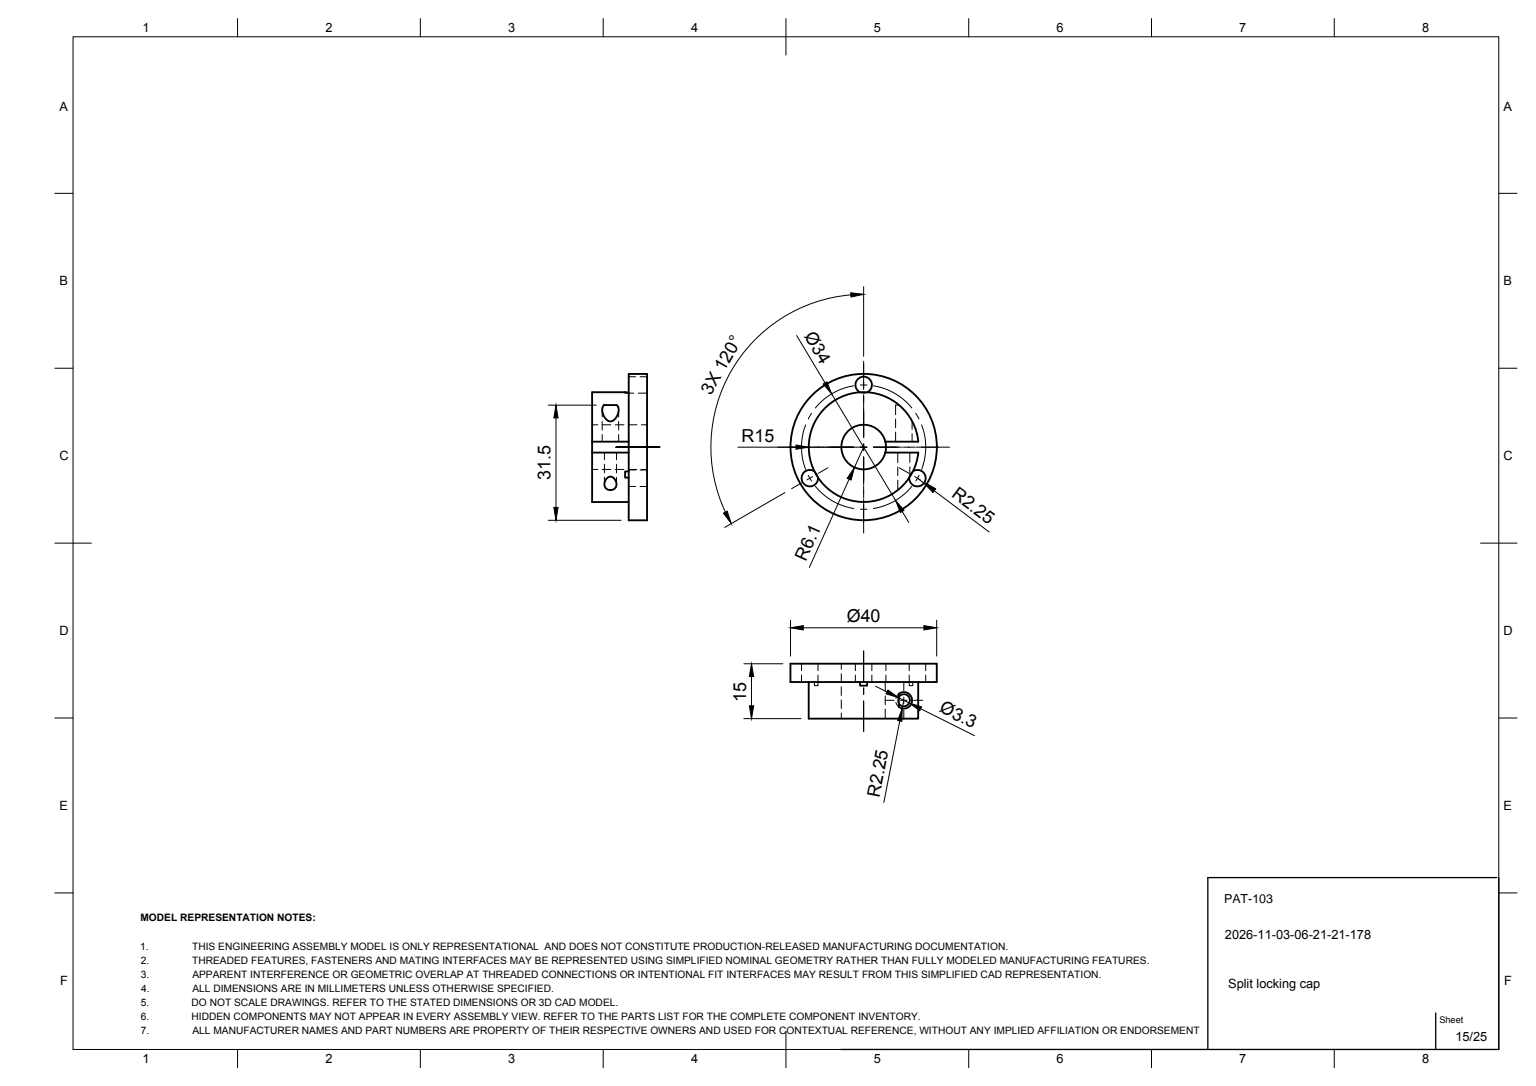
ISO-10303-21;
HEADER;
/* Generated by software containing ST-Developer
 * from STEP Tools, Inc. (www.steptools.com) 
 */

FILE_DESCRIPTION(
/* description */ ('Telescoping shaft support with lock collar'),
/* implementation_level */ '2;1');

FILE_NAME(
/* name */ 'Split locking cap.step',
/* time_stamp */ '2026-10-27T10:48:51-07:00',
/* author */ (''),
/* organization */ (''),
/* preprocessor_version */ 'ST-DEVELOPER v20.2',
/* originating_system */ 'Autodesk Translation Framework v15.17.0.0',
/* authorisation */ '');

FILE_SCHEMA (('AUTOMOTIVE_DESIGN { 1 0 10303 214 3 1 1 }'));
ENDSEC;

DATA;
#10=MECHANICAL_DESIGN_GEOMETRIC_PRESENTATION_REPRESENTATION('',(#251),#7349);
#183=B_SPLINE_CURVE_WITH_KNOTS('',3,(#6551,#6552,#6553,#6554,#6555,#6556,
#6557,#6558),.UNSPECIFIED.,.F.,.F.,(4,2,2,4),(0.211808182408868,0.240806862049815,
0.337801071942656,0.401300756844152),.UNSPECIFIED.);
#184=B_SPLINE_CURVE_WITH_KNOTS('',3,(#6559,#6560,#6561,#6562,#6563,#6564,
#6565,#6566,#6567,#6568,#6569,#6570,#6571,#6572,#6573,#6574,#6575,#6576,
#6577,#6578,#6579,#6580,#6581,#6582,#6583,#6584),.UNSPECIFIED.,.F.,.F.,
(4,2,2,2,2,2,2,2,2,2,2,2,4),(0.401300756844152,0.56115667536452,0.672834477075452,
0.784512278786384,0.830620394066968,0.876728509347553,0.922836624628137,
0.968944739908722,1.08062254161965,1.19230034333059,1.41565594675245,1.51265015664529,
1.54164883628624),.UNSPECIFIED.);
#185=B_SPLINE_CURVE_WITH_KNOTS('',3,(#6588,#6589,#6590,#6591,#6592,#6593,
#6594,#6595,#6596,#6597,#6598,#6599,#6600,#6601,#6602,#6603,#6604,#6605,
#6606,#6607,#6608,#6609,#6610,#6611,#6612,#6613,#6614,#6615,#6616,#6617),
 .UNSPECIFIED.,.F.,.F.,(4,2,2,2,2,2,2,2,2,2,2,2,2,2,4),(0.,0.0607190360347076,
0.121438072069415,0.209441873804407,0.2974456755394,0.399272742727807,0.501099809916215,
0.564787025689956,0.596630633576826,0.628474241463696,0.660317849350566,
0.692161457237437,0.755848673011177,0.857675740199585,0.959502807387993),
 .UNSPECIFIED.);
#186=B_SPLINE_CURVE_WITH_KNOTS('',3,(#6618,#6619,#6620,#6621,#6622,#6623,
#6624,#6625,#6626,#6627),.UNSPECIFIED.,.F.,.F.,(4,2,2,2,4),(0.959502807387993,
1.04750660912298,1.13551041085798,1.19622944689268,1.25694848292739),
 .UNSPECIFIED.);
#211=SHAPE_REPRESENTATION_RELATIONSHIP('SRR','None',#7453,#231);
#231=ADVANCED_BREP_SHAPE_REPRESENTATION('',(#271),#7337);
#251=STYLED_ITEM('',(#7620),#271);
#271=MANIFOLD_SOLID_BREP('Body1',#3974);
#328=FACE_BOUND('',#891,.T.);
#329=FACE_BOUND('',#892,.T.);
#330=FACE_BOUND('',#894,.T.);
#331=FACE_BOUND('',#896,.T.);
#332=FACE_BOUND('',#898,.T.);
#333=FACE_BOUND('',#903,.T.);
#334=FACE_BOUND('',#904,.T.);
#335=FACE_BOUND('',#905,.T.);
#336=FACE_BOUND('',#906,.T.);
#424=PLANE('',#4447);
#425=PLANE('',#4453);
#426=PLANE('',#4460);
#427=PLANE('',#4467);
#428=PLANE('',#4480);
#429=PLANE('',#4481);
#430=PLANE('',#4482);
#431=PLANE('',#4485);
#432=PLANE('',#4492);
#606=FACE_OUTER_BOUND('',#881,.T.);
#607=FACE_OUTER_BOUND('',#882,.T.);
#608=FACE_OUTER_BOUND('',#883,.T.);
#609=FACE_OUTER_BOUND('',#884,.T.);
#610=FACE_OUTER_BOUND('',#885,.T.);
#611=FACE_OUTER_BOUND('',#886,.T.);
#612=FACE_OUTER_BOUND('',#887,.T.);
#613=FACE_OUTER_BOUND('',#888,.T.);
#614=FACE_OUTER_BOUND('',#889,.T.);
#615=FACE_OUTER_BOUND('',#890,.T.);
#616=FACE_OUTER_BOUND('',#893,.T.);
#617=FACE_OUTER_BOUND('',#895,.T.);
#618=FACE_OUTER_BOUND('',#897,.T.);
#619=FACE_OUTER_BOUND('',#899,.T.);
#620=FACE_OUTER_BOUND('',#900,.T.);
#621=FACE_OUTER_BOUND('',#901,.T.);
#622=FACE_OUTER_BOUND('',#902,.T.);
#881=EDGE_LOOP('',(#3158,#3159));
#882=EDGE_LOOP('',(#3160,#3161,#3162,#3163,#3164,#3165));
#883=EDGE_LOOP('',(#3166,#3167,#3168,#3169,#3170));
#884=EDGE_LOOP('',(#3171,#3172));
#885=EDGE_LOOP('',(#3173,#3174,#3175,#3176,#3177,#3178,#3179,#3180));
#886=EDGE_LOOP('',(#3181,#3182));
#887=EDGE_LOOP('',(#3183,#3184,#3185,#3186,#3187,#3188,#3189,#3190));
#888=EDGE_LOOP('',(#3191,#3192));
#889=EDGE_LOOP('',(#3193,#3194,#3195,#3196,#3197,#3198,#3199,#3200));
#890=EDGE_LOOP('',(#3201,#3202,#3203,#3204,#3205,#3206,#3207,#3208,#3209,
#3210,#3211,#3212,#3213,#3214,#3215,#3216));
#891=EDGE_LOOP('',(#3217,#3218,#3219));
#892=EDGE_LOOP('',(#3220,#3221));
#893=EDGE_LOOP('',(#3222,#3223,#3224,#3225));
#894=EDGE_LOOP('',(#3226));
#895=EDGE_LOOP('',(#3227,#3228,#3229,#3230));
#896=EDGE_LOOP('',(#3231));
#897=EDGE_LOOP('',(#3232));
#898=EDGE_LOOP('',(#3233,#3234,#3235,#3236,#3237,#3238,#3239,#3240,#3241,
#3242,#3243,#3244,#3245));
#899=EDGE_LOOP('',(#3246,#3247,#3248,#3249,#3250));
#900=EDGE_LOOP('',(#3251,#3252,#3253,#3254,#3255,#3256,#3257,#3258));
#901=EDGE_LOOP('',(#3259,#3260,#3261,#3262));
#902=EDGE_LOOP('',(#3263));
#903=EDGE_LOOP('',(#3264));
#904=EDGE_LOOP('',(#3265));
#905=EDGE_LOOP('',(#3266));
#906=EDGE_LOOP('',(#3267));
#1169=LINE('',#6544,#1449);
#1170=LINE('',#6550,#1450);
#1171=LINE('',#6629,#1451);
#1172=LINE('',#6640,#1452);
#1173=LINE('',#6643,#1453);
#1174=LINE('',#6645,#1454);
#1175=LINE('',#6656,#1455);
#1176=LINE('',#6659,#1456);
#1177=LINE('',#6661,#1457);
#1178=LINE('',#6672,#1458);
#1179=LINE('',#6675,#1459);
#1180=LINE('',#6677,#1460);
#1181=LINE('',#6685,#1461);
#1182=LINE('',#6689,#1462);
#1183=LINE('',#6694,#1463);
#1184=LINE('',#6695,#1464);
#1185=LINE('',#6696,#1465);
#1186=LINE('',#6700,#1466);
#1187=LINE('',#6701,#1467);
#1188=LINE('',#6702,#1468);
#1189=LINE('',#6713,#1469);
#1190=LINE('',#6717,#1470);
#1449=VECTOR('',#5331,1.);
#1450=VECTOR('',#5338,0.225);
#1451=VECTOR('',#5341,0.164999999999999);
#1452=VECTOR('',#5354,0.225);
#1453=VECTOR('',#5357,1.);
#1454=VECTOR('',#5358,1.);
#1455=VECTOR('',#5371,0.225);
#1456=VECTOR('',#5374,1.);
#1457=VECTOR('',#5375,1.);
#1458=VECTOR('',#5388,0.225);
#1459=VECTOR('',#5391,1.);
#1460=VECTOR('',#5392,1.);
#1461=VECTOR('',#5403,1.);
#1462=VECTOR('',#5406,1.);
#1463=VECTOR('',#5411,1.);
#1464=VECTOR('',#5412,1.);
#1465=VECTOR('',#5413,1.);
#1466=VECTOR('',#5416,1.);
#1467=VECTOR('',#5417,1.);
#1468=VECTOR('',#5418,1.);
#1469=VECTOR('',#5433,0.61);
#1470=VECTOR('',#5438,2.);
#1703=CIRCLE('',#4448,0.225);
#1704=CIRCLE('',#4450,0.225);
#1705=CIRCLE('',#4452,0.164999999999999);
#1706=CIRCLE('',#4454,1.5);
#1707=CIRCLE('',#4455,0.225);
#1708=CIRCLE('',#4457,0.225);
#1709=CIRCLE('',#4458,0.225);
#1710=CIRCLE('',#4459,0.225);
#1711=CIRCLE('',#4461,1.5);
#1712=CIRCLE('',#4462,0.225);
#1713=CIRCLE('',#4464,0.225);
#1714=CIRCLE('',#4465,0.225);
#1715=CIRCLE('',#4466,0.225);
#1716=CIRCLE('',#4468,1.5);
#1717=CIRCLE('',#4469,0.225);
#1718=CIRCLE('',#4471,0.225);
#1719=CIRCLE('',#4472,0.225);
#1720=CIRCLE('',#4473,0.225);
#1721=CIRCLE('',#4475,1.5);
#1722=CIRCLE('',#4476,1.5);
#1723=CIRCLE('',#4477,1.5);
#1724=CIRCLE('',#4478,1.5);
#1725=CIRCLE('',#4479,1.5);
#1726=CIRCLE('',#4483,2.);
#1727=CIRCLE('',#4484,0.61);
#1728=CIRCLE('',#4486,0.61);
#1729=CIRCLE('',#4487,0.61);
#1730=CIRCLE('',#4489,0.61);
#1731=CIRCLE('',#4491,2.);
#1970=VERTEX_POINT('',#6542);
#1971=VERTEX_POINT('',#6543);
#1972=VERTEX_POINT('',#6547);
#1973=VERTEX_POINT('',#6549);
#1974=VERTEX_POINT('',#6586);
#1975=VERTEX_POINT('',#6587);
#1976=VERTEX_POINT('',#6628);
#1977=VERTEX_POINT('',#6632);
#1978=VERTEX_POINT('',#6633);
#1979=VERTEX_POINT('',#6637);
#1980=VERTEX_POINT('',#6639);
#1981=VERTEX_POINT('',#6641);
#1982=VERTEX_POINT('',#6644);
#1983=VERTEX_POINT('',#6648);
#1984=VERTEX_POINT('',#6649);
#1985=VERTEX_POINT('',#6653);
#1986=VERTEX_POINT('',#6655);
#1987=VERTEX_POINT('',#6657);
#1988=VERTEX_POINT('',#6660);
#1989=VERTEX_POINT('',#6664);
#1990=VERTEX_POINT('',#6665);
#1991=VERTEX_POINT('',#6669);
#1992=VERTEX_POINT('',#6671);
#1993=VERTEX_POINT('',#6673);
#1994=VERTEX_POINT('',#6676);
#1995=VERTEX_POINT('',#6682);
#1996=VERTEX_POINT('',#6684);
#1997=VERTEX_POINT('',#6686);
#1998=VERTEX_POINT('',#6688);
#1999=VERTEX_POINT('',#6692);
#2000=VERTEX_POINT('',#6693);
#2001=VERTEX_POINT('',#6698);
#2002=VERTEX_POINT('',#6699);
#2003=VERTEX_POINT('',#6704);
#2004=VERTEX_POINT('',#6708);
#2005=VERTEX_POINT('',#6712);
#2006=VERTEX_POINT('',#6716);
#2391=EDGE_CURVE('',#1970,#1971,#1169,.T.);
#2392=EDGE_CURVE('',#1971,#1970,#1703,.T.);
#2393=EDGE_CURVE('',#1972,#1972,#1704,.T.);
#2394=EDGE_CURVE('',#1972,#1973,#1170,.T.);
#2395=EDGE_CURVE('',#1971,#1973,#183,.T.);
#2396=EDGE_CURVE('',#1973,#1970,#184,.T.);
#2397=EDGE_CURVE('',#1974,#1975,#185,.T.);
#2398=EDGE_CURVE('',#1975,#1974,#186,.T.);
#2399=EDGE_CURVE('',#1975,#1976,#1171,.T.);
#2400=EDGE_CURVE('',#1976,#1976,#1705,.T.);
#2401=EDGE_CURVE('',#1977,#1978,#1706,.T.);
#2402=EDGE_CURVE('',#1978,#1977,#1707,.T.);
#2403=EDGE_CURVE('',#1979,#1979,#1708,.T.);
#2404=EDGE_CURVE('',#1979,#1980,#1172,.T.);
#2405=EDGE_CURVE('',#1981,#1980,#1709,.T.);
#2406=EDGE_CURVE('',#1978,#1981,#1173,.T.);
#2407=EDGE_CURVE('',#1982,#1977,#1174,.T.);
#2408=EDGE_CURVE('',#1980,#1982,#1710,.T.);
#2409=EDGE_CURVE('',#1983,#1984,#1711,.T.);
#2410=EDGE_CURVE('',#1984,#1983,#1712,.T.);
#2411=EDGE_CURVE('',#1985,#1985,#1713,.T.);
#2412=EDGE_CURVE('',#1985,#1986,#1175,.T.);
#2413=EDGE_CURVE('',#1987,#1986,#1714,.T.);
#2414=EDGE_CURVE('',#1984,#1987,#1176,.T.);
#2415=EDGE_CURVE('',#1988,#1983,#1177,.T.);
#2416=EDGE_CURVE('',#1986,#1988,#1715,.T.);
#2417=EDGE_CURVE('',#1989,#1990,#1716,.T.);
#2418=EDGE_CURVE('',#1990,#1989,#1717,.T.);
#2419=EDGE_CURVE('',#1991,#1991,#1718,.T.);
#2420=EDGE_CURVE('',#1991,#1992,#1178,.T.);
#2421=EDGE_CURVE('',#1993,#1992,#1719,.T.);
#2422=EDGE_CURVE('',#1990,#1993,#1179,.T.);
#2423=EDGE_CURVE('',#1994,#1989,#1180,.T.);
#2424=EDGE_CURVE('',#1992,#1994,#1720,.T.);
#2425=EDGE_CURVE('',#1988,#1981,#1721,.T.);
#2426=EDGE_CURVE('',#1994,#1987,#1722,.T.);
#2427=EDGE_CURVE('',#1995,#1993,#1723,.T.);
#2428=EDGE_CURVE('',#1995,#1996,#1181,.T.);
#2429=EDGE_CURVE('',#1997,#1996,#1724,.T.);
#2430=EDGE_CURVE('',#1997,#1998,#1182,.T.);
#2431=EDGE_CURVE('',#1982,#1998,#1725,.T.);
#2432=EDGE_CURVE('',#1999,#2000,#1183,.T.);
#2433=EDGE_CURVE('',#1998,#1999,#1184,.T.);
#2434=EDGE_CURVE('',#2000,#1997,#1185,.T.);
#2435=EDGE_CURVE('',#2001,#2002,#1186,.T.);
#2436=EDGE_CURVE('',#1996,#2001,#1187,.T.);
#2437=EDGE_CURVE('',#2002,#1995,#1188,.T.);
#2438=EDGE_CURVE('',#2003,#2003,#1726,.T.);
#2439=EDGE_CURVE('',#2002,#1999,#1727,.T.);
#2440=EDGE_CURVE('',#2001,#2004,#1728,.T.);
#2441=EDGE_CURVE('',#2004,#2000,#1729,.T.);
#2442=EDGE_CURVE('',#2004,#2005,#1189,.T.);
#2443=EDGE_CURVE('',#2005,#2005,#1730,.T.);
#2444=EDGE_CURVE('',#2003,#2006,#1190,.T.);
#2445=EDGE_CURVE('',#2006,#2006,#1731,.T.);
#3158=ORIENTED_EDGE('',*,*,#2391,.F.);
#3159=ORIENTED_EDGE('',*,*,#2392,.F.);
#3160=ORIENTED_EDGE('',*,*,#2393,.F.);
#3161=ORIENTED_EDGE('',*,*,#2394,.T.);
#3162=ORIENTED_EDGE('',*,*,#2395,.F.);
#3163=ORIENTED_EDGE('',*,*,#2392,.T.);
#3164=ORIENTED_EDGE('',*,*,#2396,.F.);
#3165=ORIENTED_EDGE('',*,*,#2394,.F.);
#3166=ORIENTED_EDGE('',*,*,#2397,.F.);
#3167=ORIENTED_EDGE('',*,*,#2398,.F.);
#3168=ORIENTED_EDGE('',*,*,#2399,.T.);
#3169=ORIENTED_EDGE('',*,*,#2400,.F.);
#3170=ORIENTED_EDGE('',*,*,#2399,.F.);
#3171=ORIENTED_EDGE('',*,*,#2401,.F.);
#3172=ORIENTED_EDGE('',*,*,#2402,.F.);
#3173=ORIENTED_EDGE('',*,*,#2403,.F.);
#3174=ORIENTED_EDGE('',*,*,#2404,.T.);
#3175=ORIENTED_EDGE('',*,*,#2405,.F.);
#3176=ORIENTED_EDGE('',*,*,#2406,.F.);
#3177=ORIENTED_EDGE('',*,*,#2402,.T.);
#3178=ORIENTED_EDGE('',*,*,#2407,.F.);
#3179=ORIENTED_EDGE('',*,*,#2408,.F.);
#3180=ORIENTED_EDGE('',*,*,#2404,.F.);
#3181=ORIENTED_EDGE('',*,*,#2409,.F.);
#3182=ORIENTED_EDGE('',*,*,#2410,.F.);
#3183=ORIENTED_EDGE('',*,*,#2411,.F.);
#3184=ORIENTED_EDGE('',*,*,#2412,.T.);
#3185=ORIENTED_EDGE('',*,*,#2413,.F.);
#3186=ORIENTED_EDGE('',*,*,#2414,.F.);
#3187=ORIENTED_EDGE('',*,*,#2410,.T.);
#3188=ORIENTED_EDGE('',*,*,#2415,.F.);
#3189=ORIENTED_EDGE('',*,*,#2416,.F.);
#3190=ORIENTED_EDGE('',*,*,#2412,.F.);
#3191=ORIENTED_EDGE('',*,*,#2417,.F.);
#3192=ORIENTED_EDGE('',*,*,#2418,.F.);
#3193=ORIENTED_EDGE('',*,*,#2419,.F.);
#3194=ORIENTED_EDGE('',*,*,#2420,.T.);
#3195=ORIENTED_EDGE('',*,*,#2421,.F.);
#3196=ORIENTED_EDGE('',*,*,#2422,.F.);
#3197=ORIENTED_EDGE('',*,*,#2418,.T.);
#3198=ORIENTED_EDGE('',*,*,#2423,.F.);
#3199=ORIENTED_EDGE('',*,*,#2424,.F.);
#3200=ORIENTED_EDGE('',*,*,#2420,.F.);
#3201=ORIENTED_EDGE('',*,*,#2407,.T.);
#3202=ORIENTED_EDGE('',*,*,#2401,.T.);
#3203=ORIENTED_EDGE('',*,*,#2406,.T.);
#3204=ORIENTED_EDGE('',*,*,#2425,.F.);
#3205=ORIENTED_EDGE('',*,*,#2415,.T.);
#3206=ORIENTED_EDGE('',*,*,#2409,.T.);
#3207=ORIENTED_EDGE('',*,*,#2414,.T.);
#3208=ORIENTED_EDGE('',*,*,#2426,.F.);
#3209=ORIENTED_EDGE('',*,*,#2423,.T.);
#3210=ORIENTED_EDGE('',*,*,#2417,.T.);
#3211=ORIENTED_EDGE('',*,*,#2422,.T.);
#3212=ORIENTED_EDGE('',*,*,#2427,.F.);
#3213=ORIENTED_EDGE('',*,*,#2428,.T.);
#3214=ORIENTED_EDGE('',*,*,#2429,.F.);
#3215=ORIENTED_EDGE('',*,*,#2430,.T.);
#3216=ORIENTED_EDGE('',*,*,#2431,.F.);
#3217=ORIENTED_EDGE('',*,*,#2395,.T.);
#3218=ORIENTED_EDGE('',*,*,#2396,.T.);
#3219=ORIENTED_EDGE('',*,*,#2391,.T.);
#3220=ORIENTED_EDGE('',*,*,#2397,.T.);
#3221=ORIENTED_EDGE('',*,*,#2398,.T.);
#3222=ORIENTED_EDGE('',*,*,#2432,.F.);
#3223=ORIENTED_EDGE('',*,*,#2433,.F.);
#3224=ORIENTED_EDGE('',*,*,#2430,.F.);
#3225=ORIENTED_EDGE('',*,*,#2434,.F.);
#3226=ORIENTED_EDGE('',*,*,#2393,.T.);
#3227=ORIENTED_EDGE('',*,*,#2435,.F.);
#3228=ORIENTED_EDGE('',*,*,#2436,.F.);
#3229=ORIENTED_EDGE('',*,*,#2428,.F.);
#3230=ORIENTED_EDGE('',*,*,#2437,.F.);
#3231=ORIENTED_EDGE('',*,*,#2400,.T.);
#3232=ORIENTED_EDGE('',*,*,#2438,.T.);
#3233=ORIENTED_EDGE('',*,*,#2405,.T.);
#3234=ORIENTED_EDGE('',*,*,#2408,.T.);
#3235=ORIENTED_EDGE('',*,*,#2431,.T.);
#3236=ORIENTED_EDGE('',*,*,#2433,.T.);
#3237=ORIENTED_EDGE('',*,*,#2439,.F.);
#3238=ORIENTED_EDGE('',*,*,#2437,.T.);
#3239=ORIENTED_EDGE('',*,*,#2427,.T.);
#3240=ORIENTED_EDGE('',*,*,#2421,.T.);
#3241=ORIENTED_EDGE('',*,*,#2424,.T.);
#3242=ORIENTED_EDGE('',*,*,#2426,.T.);
#3243=ORIENTED_EDGE('',*,*,#2413,.T.);
#3244=ORIENTED_EDGE('',*,*,#2416,.T.);
#3245=ORIENTED_EDGE('',*,*,#2425,.T.);
#3246=ORIENTED_EDGE('',*,*,#2434,.T.);
#3247=ORIENTED_EDGE('',*,*,#2429,.T.);
#3248=ORIENTED_EDGE('',*,*,#2436,.T.);
#3249=ORIENTED_EDGE('',*,*,#2440,.T.);
#3250=ORIENTED_EDGE('',*,*,#2441,.T.);
#3251=ORIENTED_EDGE('',*,*,#2432,.T.);
#3252=ORIENTED_EDGE('',*,*,#2441,.F.);
#3253=ORIENTED_EDGE('',*,*,#2442,.T.);
#3254=ORIENTED_EDGE('',*,*,#2443,.T.);
#3255=ORIENTED_EDGE('',*,*,#2442,.F.);
#3256=ORIENTED_EDGE('',*,*,#2440,.F.);
#3257=ORIENTED_EDGE('',*,*,#2435,.T.);
#3258=ORIENTED_EDGE('',*,*,#2439,.T.);
#3259=ORIENTED_EDGE('',*,*,#2438,.F.);
#3260=ORIENTED_EDGE('',*,*,#2444,.T.);
#3261=ORIENTED_EDGE('',*,*,#2445,.T.);
#3262=ORIENTED_EDGE('',*,*,#2444,.F.);
#3263=ORIENTED_EDGE('',*,*,#2445,.F.);
#3264=ORIENTED_EDGE('',*,*,#2403,.T.);
#3265=ORIENTED_EDGE('',*,*,#2411,.T.);
#3266=ORIENTED_EDGE('',*,*,#2419,.T.);
#3267=ORIENTED_EDGE('',*,*,#2443,.F.);
#3706=CYLINDRICAL_SURFACE('',#4449,0.225);
#3707=CYLINDRICAL_SURFACE('',#4451,0.164999999999999);
#3708=CYLINDRICAL_SURFACE('',#4456,0.225);
#3709=CYLINDRICAL_SURFACE('',#4463,0.225);
#3710=CYLINDRICAL_SURFACE('',#4470,0.225);
#3711=CYLINDRICAL_SURFACE('',#4474,1.5);
#3712=CYLINDRICAL_SURFACE('',#4488,0.61);
#3713=CYLINDRICAL_SURFACE('',#4490,2.);
#3849=ADVANCED_FACE('',(#606),#424,.F.);
#3850=ADVANCED_FACE('',(#607),#3706,.F.);
#3851=ADVANCED_FACE('',(#608),#3707,.F.);
#3852=ADVANCED_FACE('',(#609),#425,.F.);
#3853=ADVANCED_FACE('',(#610),#3708,.F.);
#3854=ADVANCED_FACE('',(#611),#426,.F.);
#3855=ADVANCED_FACE('',(#612),#3709,.F.);
#3856=ADVANCED_FACE('',(#613),#427,.F.);
#3857=ADVANCED_FACE('',(#614),#3710,.F.);
#3858=ADVANCED_FACE('',(#615,#328,#329),#3711,.T.);
#3859=ADVANCED_FACE('',(#616,#330),#428,.F.);
#3860=ADVANCED_FACE('',(#617,#331),#429,.F.);
#3861=ADVANCED_FACE('',(#618,#332),#430,.T.);
#3862=ADVANCED_FACE('',(#619),#431,.T.);
#3863=ADVANCED_FACE('',(#620),#3712,.F.);
#3864=ADVANCED_FACE('',(#621),#3713,.T.);
#3865=ADVANCED_FACE('',(#622,#333,#334,#335,#336),#432,.F.);
#3974=CLOSED_SHELL('',(#3849,#3850,#3851,#3852,#3853,#3854,#3855,#3856,
#3857,#3858,#3859,#3860,#3861,#3862,#3863,#3864,#3865));
#4446=AXIS2_PLACEMENT_3D('',#6540,#5327,#5328);
#4447=AXIS2_PLACEMENT_3D('',#6541,#5329,#5330);
#4448=AXIS2_PLACEMENT_3D('',#6545,#5332,#5333);
#4449=AXIS2_PLACEMENT_3D('',#6546,#5334,#5335);
#4450=AXIS2_PLACEMENT_3D('',#6548,#5336,#5337);
#4451=AXIS2_PLACEMENT_3D('',#6585,#5339,#5340);
#4452=AXIS2_PLACEMENT_3D('',#6630,#5342,#5343);
#4453=AXIS2_PLACEMENT_3D('',#6631,#5344,#5345);
#4454=AXIS2_PLACEMENT_3D('',#6634,#5346,#5347);
#4455=AXIS2_PLACEMENT_3D('',#6635,#5348,#5349);
#4456=AXIS2_PLACEMENT_3D('',#6636,#5350,#5351);
#4457=AXIS2_PLACEMENT_3D('',#6638,#5352,#5353);
#4458=AXIS2_PLACEMENT_3D('',#6642,#5355,#5356);
#4459=AXIS2_PLACEMENT_3D('',#6646,#5359,#5360);
#4460=AXIS2_PLACEMENT_3D('',#6647,#5361,#5362);
#4461=AXIS2_PLACEMENT_3D('',#6650,#5363,#5364);
#4462=AXIS2_PLACEMENT_3D('',#6651,#5365,#5366);
#4463=AXIS2_PLACEMENT_3D('',#6652,#5367,#5368);
#4464=AXIS2_PLACEMENT_3D('',#6654,#5369,#5370);
#4465=AXIS2_PLACEMENT_3D('',#6658,#5372,#5373);
#4466=AXIS2_PLACEMENT_3D('',#6662,#5376,#5377);
#4467=AXIS2_PLACEMENT_3D('',#6663,#5378,#5379);
#4468=AXIS2_PLACEMENT_3D('',#6666,#5380,#5381);
#4469=AXIS2_PLACEMENT_3D('',#6667,#5382,#5383);
#4470=AXIS2_PLACEMENT_3D('',#6668,#5384,#5385);
#4471=AXIS2_PLACEMENT_3D('',#6670,#5386,#5387);
#4472=AXIS2_PLACEMENT_3D('',#6674,#5389,#5390);
#4473=AXIS2_PLACEMENT_3D('',#6678,#5393,#5394);
#4474=AXIS2_PLACEMENT_3D('',#6679,#5395,#5396);
#4475=AXIS2_PLACEMENT_3D('',#6680,#5397,#5398);
#4476=AXIS2_PLACEMENT_3D('',#6681,#5399,#5400);
#4477=AXIS2_PLACEMENT_3D('',#6683,#5401,#5402);
#4478=AXIS2_PLACEMENT_3D('',#6687,#5404,#5405);
#4479=AXIS2_PLACEMENT_3D('',#6690,#5407,#5408);
#4480=AXIS2_PLACEMENT_3D('',#6691,#5409,#5410);
#4481=AXIS2_PLACEMENT_3D('',#6697,#5414,#5415);
#4482=AXIS2_PLACEMENT_3D('',#6703,#5419,#5420);
#4483=AXIS2_PLACEMENT_3D('',#6705,#5421,#5422);
#4484=AXIS2_PLACEMENT_3D('',#6706,#5423,#5424);
#4485=AXIS2_PLACEMENT_3D('',#6707,#5425,#5426);
#4486=AXIS2_PLACEMENT_3D('',#6709,#5427,#5428);
#4487=AXIS2_PLACEMENT_3D('',#6710,#5429,#5430);
#4488=AXIS2_PLACEMENT_3D('',#6711,#5431,#5432);
#4489=AXIS2_PLACEMENT_3D('',#6714,#5434,#5435);
#4490=AXIS2_PLACEMENT_3D('',#6715,#5436,#5437);
#4491=AXIS2_PLACEMENT_3D('',#6718,#5439,#5440);
#4492=AXIS2_PLACEMENT_3D('',#6719,#5441,#5442);
#5327=DIRECTION('axis',(0.,0.,1.));
#5328=DIRECTION('refdir',(1.,0.,0.));
#5329=DIRECTION('center_axis',(0.,0.,1.));
#5330=DIRECTION('ref_axis',(1.,0.,0.));
#5331=DIRECTION('',(-1.,0.,0.));
#5332=DIRECTION('center_axis',(0.,0.,1.));
#5333=DIRECTION('ref_axis',(1.,0.,0.));
#5334=DIRECTION('center_axis',(0.,0.,1.));
#5335=DIRECTION('ref_axis',(1.,0.,0.));
#5336=DIRECTION('center_axis',(0.,0.,1.));
#5337=DIRECTION('ref_axis',(1.,0.,0.));
#5338=DIRECTION('',(0.,0.,1.));
#5339=DIRECTION('center_axis',(0.,0.,1.));
#5340=DIRECTION('ref_axis',(1.,0.,0.));
#5341=DIRECTION('',(0.,0.,1.));
#5342=DIRECTION('center_axis',(0.,0.,-1.));
#5343=DIRECTION('ref_axis',(1.,0.,0.));
#5344=DIRECTION('center_axis',(1.,0.,0.));
#5345=DIRECTION('ref_axis',(0.,0.,-1.));
#5346=DIRECTION('center_axis',(1.,0.,0.));
#5347=DIRECTION('ref_axis',(0.,0.,-1.));
#5348=DIRECTION('center_axis',(1.,0.,0.));
#5349=DIRECTION('ref_axis',(0.,0.,-1.));
#5350=DIRECTION('center_axis',(1.,0.,0.));
#5351=DIRECTION('ref_axis',(0.,0.,-1.));
#5352=DIRECTION('center_axis',(1.,0.,0.));
#5353=DIRECTION('ref_axis',(0.,0.,-1.));
#5354=DIRECTION('',(1.,0.,0.));
#5355=DIRECTION('center_axis',(-1.,0.,0.));
#5356=DIRECTION('ref_axis',(0.,0.,-1.));
#5357=DIRECTION('',(-1.,0.,0.));
#5358=DIRECTION('',(1.,0.,0.));
#5359=DIRECTION('center_axis',(-1.,0.,0.));
#5360=DIRECTION('ref_axis',(0.,0.,-1.));
#5361=DIRECTION('center_axis',(1.,0.,0.));
#5362=DIRECTION('ref_axis',(0.,0.,-1.));
#5363=DIRECTION('center_axis',(1.,0.,0.));
#5364=DIRECTION('ref_axis',(0.,0.,-1.));
#5365=DIRECTION('center_axis',(1.,0.,0.));
#5366=DIRECTION('ref_axis',(0.,0.,-1.));
#5367=DIRECTION('center_axis',(1.,0.,0.));
#5368=DIRECTION('ref_axis',(0.,0.,-1.));
#5369=DIRECTION('center_axis',(1.,0.,0.));
#5370=DIRECTION('ref_axis',(0.,0.,-1.));
#5371=DIRECTION('',(1.,0.,0.));
#5372=DIRECTION('center_axis',(-1.,0.,0.));
#5373=DIRECTION('ref_axis',(0.,0.,-1.));
#5374=DIRECTION('',(-1.,0.,0.));
#5375=DIRECTION('',(1.,0.,0.));
#5376=DIRECTION('center_axis',(-1.,0.,0.));
#5377=DIRECTION('ref_axis',(0.,0.,-1.));
#5378=DIRECTION('center_axis',(1.,0.,0.));
#5379=DIRECTION('ref_axis',(0.,0.,-1.));
#5380=DIRECTION('center_axis',(1.,0.,0.));
#5381=DIRECTION('ref_axis',(0.,0.,-1.));
#5382=DIRECTION('center_axis',(1.,0.,0.));
#5383=DIRECTION('ref_axis',(0.,0.,-1.));
#5384=DIRECTION('center_axis',(1.,0.,0.));
#5385=DIRECTION('ref_axis',(0.,0.,-1.));
#5386=DIRECTION('center_axis',(1.,0.,0.));
#5387=DIRECTION('ref_axis',(0.,0.,-1.));
#5388=DIRECTION('',(1.,0.,0.));
#5389=DIRECTION('center_axis',(-1.,0.,0.));
#5390=DIRECTION('ref_axis',(0.,0.,-1.));
#5391=DIRECTION('',(-1.,0.,0.));
#5392=DIRECTION('',(1.,0.,0.));
#5393=DIRECTION('center_axis',(-1.,0.,0.));
#5394=DIRECTION('ref_axis',(0.,0.,-1.));
#5395=DIRECTION('center_axis',(1.,0.,0.));
#5396=DIRECTION('ref_axis',(0.,-1.,1.83697019872103E-16));
#5397=DIRECTION('center_axis',(-1.,0.,0.));
#5398=DIRECTION('ref_axis',(0.,0.,-1.));
#5399=DIRECTION('center_axis',(-1.,0.,0.));
#5400=DIRECTION('ref_axis',(0.,0.,-1.));
#5401=DIRECTION('center_axis',(-1.,0.,0.));
#5402=DIRECTION('ref_axis',(0.,0.,-1.));
#5403=DIRECTION('',(1.,0.,0.));
#5404=DIRECTION('center_axis',(1.,0.,0.));
#5405=DIRECTION('ref_axis',(0.,0.,-1.));
#5406=DIRECTION('',(-1.,0.,0.));
#5407=DIRECTION('center_axis',(-1.,0.,0.));
#5408=DIRECTION('ref_axis',(0.,0.,-1.));
#5409=DIRECTION('center_axis',(0.,0.,1.));
#5410=DIRECTION('ref_axis',(0.,-1.,0.));
#5411=DIRECTION('',(1.,0.,0.));
#5412=DIRECTION('',(0.,-1.,0.));
#5413=DIRECTION('',(0.,1.,0.));
#5414=DIRECTION('center_axis',(0.,0.,-1.));
#5415=DIRECTION('ref_axis',(0.,1.,0.));
#5416=DIRECTION('',(-1.,0.,0.));
#5417=DIRECTION('',(0.,-1.,0.));
#5418=DIRECTION('',(0.,1.,0.));
#5419=DIRECTION('center_axis',(1.,0.,0.));
#5420=DIRECTION('ref_axis',(0.,0.,-1.));
#5421=DIRECTION('center_axis',(1.,0.,0.));
#5422=DIRECTION('ref_axis',(0.,0.,-1.));
#5423=DIRECTION('center_axis',(1.,0.,0.));
#5424=DIRECTION('ref_axis',(0.,0.,-1.));
#5425=DIRECTION('center_axis',(1.,0.,0.));
#5426=DIRECTION('ref_axis',(0.,0.,-1.));
#5427=DIRECTION('center_axis',(-1.,0.,0.));
#5428=DIRECTION('ref_axis',(0.,0.,-1.));
#5429=DIRECTION('center_axis',(-1.,0.,0.));
#5430=DIRECTION('ref_axis',(0.,0.,-1.));
#5431=DIRECTION('center_axis',(1.,0.,0.));
#5432=DIRECTION('ref_axis',(0.,0.,-1.));
#5433=DIRECTION('',(-1.,0.,0.));
#5434=DIRECTION('center_axis',(-1.,0.,0.));
#5435=DIRECTION('ref_axis',(0.,0.,-1.));
#5436=DIRECTION('center_axis',(1.,0.,0.));
#5437=DIRECTION('ref_axis',(0.,0.,-1.));
#5438=DIRECTION('',(-1.,0.,0.));
#5439=DIRECTION('center_axis',(1.,0.,0.));
#5440=DIRECTION('ref_axis',(0.,0.,-1.));
#5441=DIRECTION('center_axis',(1.,0.,0.));
#5442=DIRECTION('ref_axis',(0.,0.,-1.));
#6540=CARTESIAN_POINT('',(0.,0.,0.));
#6541=CARTESIAN_POINT('Origin',(11.,1.1,4.65));
#6542=CARTESIAN_POINT('',(11.1785346780556,0.963068014212911,4.65));
#6543=CARTESIAN_POINT('',(10.8214653219444,0.963068014212911,4.65));
#6544=CARTESIAN_POINT('',(10.5,0.963068014212911,4.65));
#6545=CARTESIAN_POINT('Origin',(11.,1.1,4.65));
#6546=CARTESIAN_POINT('Origin',(11.,1.1,3.65));
#6547=CARTESIAN_POINT('',(10.775,1.1,3.65));
#6548=CARTESIAN_POINT('Origin',(11.,1.1,3.65));
#6549=CARTESIAN_POINT('',(10.775,1.09999999957979,4.51980390362508));
#6550=CARTESIAN_POINT('',(10.775,1.1,3.65));
#6551=CARTESIAN_POINT('Ctrl Pts',(10.8214653219444,0.963068014212911,4.65));
#6552=CARTESIAN_POINT('Ctrl Pts',(10.8162688127795,0.969843327412709,4.6443260109313));
#6553=CARTESIAN_POINT('Ctrl Pts',(10.8115201211091,0.976836537416272,4.63836687623802));
#6554=CARTESIAN_POINT('Ctrl Pts',(10.792918343781,1.0077339139021,4.61151493738561));
#6555=CARTESIAN_POINT('Ctrl Pts',(10.7840010147256,1.03286247939125,4.58821848420302));
#6556=CARTESIAN_POINT('Ctrl Pts',(10.7764275645432,1.07048803422142,4.55094929145805));
#6557=CARTESIAN_POINT('Ctrl Pts',(10.7750000000547,1.08535718524001,4.53559821000295));
#6558=CARTESIAN_POINT('Ctrl Pts',(10.775,1.09999999915957,4.51980390362508));
#6559=CARTESIAN_POINT('Ctrl Pts',(10.775,1.09999999915957,4.51980390362508));
#6560=CARTESIAN_POINT('Ctrl Pts',(10.7749999998623,1.13686223670398,4.48004286611214));
#6561=CARTESIAN_POINT('Ctrl Pts',(10.7839934300633,1.17220221216353,4.4373912158357));
#6562=CARTESIAN_POINT('Ctrl Pts',(10.8116025036461,1.22546035116394,4.36579074537975));
#6563=CARTESIAN_POINT('Ctrl Pts',(10.826392404746,1.24536021423858,4.33673835178744));
#6564=CARTESIAN_POINT('Ctrl Pts',(10.8631377994706,1.28038279168244,4.28209526166438));
#6565=CARTESIAN_POINT('Ctrl Pts',(10.8846693973938,1.29561277550653,4.25628935065431));
#6566=CARTESIAN_POINT('Ctrl Pts',(10.9246244306808,1.31237665040526,4.22647603162929));
#6567=CARTESIAN_POINT('Ctrl Pts',(10.9385046923607,1.3169746204353,4.21806846608269));
#6568=CARTESIAN_POINT('Ctrl Pts',(10.9684801775212,1.32330731829159,4.20633010315014));
#6569=CARTESIAN_POINT('Ctrl Pts',(10.9846306282398,1.325,4.20311805552126));
#6570=CARTESIAN_POINT('Ctrl Pts',(11.0153693717602,1.325,4.20311805552126));
#6571=CARTESIAN_POINT('Ctrl Pts',(11.0315198224788,1.32330731829159,4.20633010315014));
#6572=CARTESIAN_POINT('Ctrl Pts',(11.0614953076393,1.3169746204353,4.21806846608269));
#6573=CARTESIAN_POINT('Ctrl Pts',(11.0753755693192,1.31237665040526,4.22647603162929));
#6574=CARTESIAN_POINT('Ctrl Pts',(11.1153306026062,1.29561277550653,4.25628935065431));
#6575=CARTESIAN_POINT('Ctrl Pts',(11.1368622005294,1.28038279168244,4.28209526166438));
#6576=CARTESIAN_POINT('Ctrl Pts',(11.173607595254,1.24536021423858,4.33673835178744));
#6577=CARTESIAN_POINT('Ctrl Pts',(11.1883974963539,1.22546035116394,4.36579074537975));
#6578=CARTESIAN_POINT('Ctrl Pts',(11.222463106795,1.15974749736021,4.45413538782613));
#6579=CARTESIAN_POINT('Ctrl Pts',(11.2311157805594,1.10796402441359,4.51382824678284));
#6580=CARTESIAN_POINT('Ctrl Pts',(11.2159989852744,1.03286247939125,4.58821848420302));
#6581=CARTESIAN_POINT('Ctrl Pts',(11.207081656219,1.0077339139021,4.61151493738561));
#6582=CARTESIAN_POINT('Ctrl Pts',(11.1884798788909,0.976836537416272,4.63836687623803));
#6583=CARTESIAN_POINT('Ctrl Pts',(11.1837311872205,0.969843327412708,4.64432601093131));
#6584=CARTESIAN_POINT('Ctrl Pts',(11.1785346780556,0.963068014212911,4.65));
#6585=CARTESIAN_POINT('Origin',(11.,1.1,2.3));
#6586=CARTESIAN_POINT('',(11.,0.935000000000001,2.32706564548565));
#6587=CARTESIAN_POINT('',(10.835,1.1,2.48019609728144));
#6588=CARTESIAN_POINT('Ctrl Pts',(11.,0.935000000000001,2.32706564548565));
#6589=CARTESIAN_POINT('Ctrl Pts',(11.0202396786782,0.935000000000001,2.32706564548565));
#6590=CARTESIAN_POINT('Ctrl Pts',(11.0413998843664,0.938976037222427,2.33020641131557));
#6591=CARTESIAN_POINT('Ctrl Pts',(11.079434847611,0.953942593189685,2.34237891599741));
#6592=CARTESIAN_POINT('Ctrl Pts',(11.0963248656201,0.964885450235815,2.35142151909605));
#6593=CARTESIAN_POINT('Ctrl Pts',(11.1285584673749,0.993474390588197,2.3759424605798));
#6594=CARTESIAN_POINT('Ctrl Pts',(11.142996001906,1.01439122017948,2.39460099158616));
#6595=CARTESIAN_POINT('Ctrl Pts',(11.161205098565,1.0576959560997,2.43596250694638));
#6596=CARTESIAN_POINT('Ctrl Pts',(11.165,1.08005630656369,2.45868405685733));
#6597=CARTESIAN_POINT('Ctrl Pts',(11.165,1.12307636456025,2.50508715814972));
#6598=CARTESIAN_POINT('Ctrl Pts',(11.1599788863536,1.14709181073674,2.53283337360734));
#6599=CARTESIAN_POINT('Ctrl Pts',(11.1397130351965,1.19105576310235,2.58752146760594));
#6600=CARTESIAN_POINT('Ctrl Pts',(11.1246027452831,1.21104555821498,2.61447988461167));
#6601=CARTESIAN_POINT('Ctrl Pts',(11.0931318205307,1.23710826004727,2.65155012736531));
#6602=CARTESIAN_POINT('Ctrl Pts',(11.0776964270187,1.24683112690748,2.6659894549942));
#6603=CARTESIAN_POINT('Ctrl Pts',(11.0507603369974,1.25729325232077,2.68192051821757));
#6604=CARTESIAN_POINT('Ctrl Pts',(11.0411497301163,1.2601136995706,2.68628885375725));
#6605=CARTESIAN_POINT('Ctrl Pts',(11.0210767897834,1.26396632271753,2.69228583186432));
#6606=CARTESIAN_POINT('Ctrl Pts',(11.0106145359623,1.265,2.69391377632414));
#6607=CARTESIAN_POINT('Ctrl Pts',(10.9893854640377,1.265,2.69391377632414));
#6608=CARTESIAN_POINT('Ctrl Pts',(10.9789232102166,1.26396632271753,2.69228583186432));
#6609=CARTESIAN_POINT('Ctrl Pts',(10.9588502698837,1.2601136995706,2.68628885375725));
#6610=CARTESIAN_POINT('Ctrl Pts',(10.9492396630026,1.25729325232077,2.68192051821757));
#6611=CARTESIAN_POINT('Ctrl Pts',(10.9223035729813,1.24683112690748,2.6659894549942));
#6612=CARTESIAN_POINT('Ctrl Pts',(10.9068681794693,1.23710826004727,2.65155012736531));
#6613=CARTESIAN_POINT('Ctrl Pts',(10.8753972547169,1.21104555821498,2.61447988461167));
#6614=CARTESIAN_POINT('Ctrl Pts',(10.8602869648035,1.19105576310235,2.58752146760594));
#6615=CARTESIAN_POINT('Ctrl Pts',(10.8400211136464,1.14709181073674,2.53283337360734));
#6616=CARTESIAN_POINT('Ctrl Pts',(10.835,1.12307636456025,2.50508715814972));
#6617=CARTESIAN_POINT('Ctrl Pts',(10.835,1.1,2.48019609728144));
#6618=CARTESIAN_POINT('Ctrl Pts',(10.835,1.1,2.48019609728144));
#6619=CARTESIAN_POINT('Ctrl Pts',(10.835,1.08005630656369,2.45868405685733));
#6620=CARTESIAN_POINT('Ctrl Pts',(10.838794901435,1.0576959560997,2.43596250694638));
#6621=CARTESIAN_POINT('Ctrl Pts',(10.857003998094,1.01439122017948,2.39460099158616));
#6622=CARTESIAN_POINT('Ctrl Pts',(10.8714415326251,0.993474390588197,2.3759424605798));
#6623=CARTESIAN_POINT('Ctrl Pts',(10.9036751343799,0.964885450235815,2.35142151909605));
#6624=CARTESIAN_POINT('Ctrl Pts',(10.920565152389,0.953942593189685,2.34237891599741));
#6625=CARTESIAN_POINT('Ctrl Pts',(10.9586001156336,0.938976037222427,2.33020641131557));
#6626=CARTESIAN_POINT('Ctrl Pts',(10.9797603213218,0.935000000000001,2.32706564548565));
#6627=CARTESIAN_POINT('Ctrl Pts',(11.,0.935000000000001,2.32706564548565));
#6628=CARTESIAN_POINT('',(10.835,1.1,3.35));
#6629=CARTESIAN_POINT('',(10.835,1.1,2.3));
#6630=CARTESIAN_POINT('Origin',(11.,1.1,3.35));
#6631=CARTESIAN_POINT('Origin',(10.6,1.11022302462516E-16,5.2));
#6632=CARTESIAN_POINT('',(10.6,0.0967741410450116,4.996875));
#6633=CARTESIAN_POINT('',(10.6,-0.0967741410450114,4.996875));
#6634=CARTESIAN_POINT('Origin',(10.6,0.,3.5));
#6635=CARTESIAN_POINT('Origin',(10.6,1.04094977927525E-16,5.2));
#6636=CARTESIAN_POINT('Origin',(9.9,1.04094977927525E-16,5.2));
#6637=CARTESIAN_POINT('',(10.,7.65404249467096E-17,5.425));
#6638=CARTESIAN_POINT('Origin',(10.,1.04094977927525E-16,5.2));
#6639=CARTESIAN_POINT('',(10.5,7.65404249467096E-17,5.425));
#6640=CARTESIAN_POINT('',(9.9,7.65404249467096E-17,5.425));
#6641=CARTESIAN_POINT('',(10.5,-0.0967741410450087,4.996875));
#6642=CARTESIAN_POINT('Origin',(10.5,1.04094977927525E-16,5.2));
#6643=CARTESIAN_POINT('',(9.9,-0.0967741410450114,4.996875));
#6644=CARTESIAN_POINT('',(10.5,0.0967741410450089,4.996875));
#6645=CARTESIAN_POINT('',(9.9,0.0967741410450116,4.996875));
#6646=CARTESIAN_POINT('Origin',(10.5,1.04094977927525E-16,5.2));
#6647=CARTESIAN_POINT('Origin',(10.6,-1.47224318643355,2.65));
#6648=CARTESIAN_POINT('',(10.6,-1.34471884681234,2.8353713645744));
#6649=CARTESIAN_POINT('',(10.6,-1.24794470576733,2.6677536354256));
#6650=CARTESIAN_POINT('Origin',(10.6,0.,3.5));
#6651=CARTESIAN_POINT('Origin',(10.6,-1.47224318643355,2.65));
#6652=CARTESIAN_POINT('Origin',(9.9,-1.47224318643355,2.65));
#6653=CARTESIAN_POINT('',(10.,-1.47224318643355,2.875));
#6654=CARTESIAN_POINT('Origin',(10.,-1.47224318643355,2.65));
#6655=CARTESIAN_POINT('',(10.5,-1.47224318643355,2.875));
#6656=CARTESIAN_POINT('',(9.9,-1.47224318643355,2.875));
#6657=CARTESIAN_POINT('',(10.5,-1.24794470576732,2.6677536354256));
#6658=CARTESIAN_POINT('Origin',(10.5,-1.47224318643355,2.65));
#6659=CARTESIAN_POINT('',(9.9,-1.24794470576733,2.6677536354256));
#6660=CARTESIAN_POINT('',(10.5,-1.34471884681234,2.8353713645744));
#6661=CARTESIAN_POINT('',(9.9,-1.34471884681234,2.8353713645744));
#6662=CARTESIAN_POINT('Origin',(10.5,-1.47224318643355,2.65));
#6663=CARTESIAN_POINT('Origin',(10.6,1.47224318643355,2.65));
#6664=CARTESIAN_POINT('',(10.6,1.24794470576732,2.6677536354256));
#6665=CARTESIAN_POINT('',(10.6,1.34471884681234,2.8353713645744));
#6666=CARTESIAN_POINT('Origin',(10.6,0.,3.5));
#6667=CARTESIAN_POINT('Origin',(10.6,1.47224318643355,2.65));
#6668=CARTESIAN_POINT('Origin',(9.9,1.47224318643355,2.65));
#6669=CARTESIAN_POINT('',(10.,1.47224318643355,2.875));
#6670=CARTESIAN_POINT('Origin',(10.,1.47224318643355,2.65));
#6671=CARTESIAN_POINT('',(10.5,1.47224318643355,2.875));
#6672=CARTESIAN_POINT('',(9.9,1.47224318643355,2.875));
#6673=CARTESIAN_POINT('',(10.5,1.34471884681234,2.8353713645744));
#6674=CARTESIAN_POINT('Origin',(10.5,1.47224318643355,2.65));
#6675=CARTESIAN_POINT('',(9.9,1.34471884681234,2.8353713645744));
#6676=CARTESIAN_POINT('',(10.5,1.24794470576732,2.6677536354256));
#6677=CARTESIAN_POINT('',(9.9,1.24794470576732,2.6677536354256));
#6678=CARTESIAN_POINT('Origin',(10.5,1.47224318643355,2.65));
#6679=CARTESIAN_POINT('Origin',(10.5,0.,3.5));
#6680=CARTESIAN_POINT('Origin',(10.5,0.,3.5));
#6681=CARTESIAN_POINT('Origin',(10.5,0.,3.5));
#6682=CARTESIAN_POINT('',(10.5,1.49248115565993,3.35));
#6683=CARTESIAN_POINT('Origin',(10.5,0.,3.5));
#6684=CARTESIAN_POINT('',(11.5,1.49248115565993,3.35));
#6685=CARTESIAN_POINT('',(10.5,1.49248115565993,3.35));
#6686=CARTESIAN_POINT('',(11.5,1.49248115565993,3.65));
#6687=CARTESIAN_POINT('Origin',(11.5,0.,3.5));
#6688=CARTESIAN_POINT('',(10.5,1.49248115565993,3.65));
#6689=CARTESIAN_POINT('',(10.5,1.49248115565993,3.65));
#6690=CARTESIAN_POINT('Origin',(10.5,0.,3.5));
#6691=CARTESIAN_POINT('Origin',(10.5,1.6,3.65));
#6692=CARTESIAN_POINT('',(10.5,0.591269819963779,3.65));
#6693=CARTESIAN_POINT('',(11.5,0.591269819963779,3.65));
#6694=CARTESIAN_POINT('',(10.,0.591269819963779,3.65));
#6695=CARTESIAN_POINT('',(10.5,1.6,3.65));
#6696=CARTESIAN_POINT('',(11.5,0.8,3.65));
#6697=CARTESIAN_POINT('Origin',(10.5,0.,3.35));
#6698=CARTESIAN_POINT('',(11.5,0.591269819963779,3.35));
#6699=CARTESIAN_POINT('',(10.5,0.591269819963779,3.35));
#6700=CARTESIAN_POINT('',(10.,0.591269819963779,3.35));
#6701=CARTESIAN_POINT('',(11.5,0.,3.35));
#6702=CARTESIAN_POINT('',(10.5,0.,3.35));
#6703=CARTESIAN_POINT('Origin',(10.5,0.,3.5));
#6704=CARTESIAN_POINT('',(10.5,-2.44929359829471E-16,5.5));
#6705=CARTESIAN_POINT('Origin',(10.5,0.,3.5));
#6706=CARTESIAN_POINT('Origin',(10.5,0.,3.5));
#6707=CARTESIAN_POINT('Origin',(11.5,0.,3.5));
#6708=CARTESIAN_POINT('',(11.5,-7.47034547479885E-17,4.11));
#6709=CARTESIAN_POINT('Origin',(11.5,0.,3.5));
#6710=CARTESIAN_POINT('Origin',(11.5,0.,3.5));
#6711=CARTESIAN_POINT('Origin',(10.,0.,3.5));
#6712=CARTESIAN_POINT('',(10.,-7.47034547479885E-17,4.11));
#6713=CARTESIAN_POINT('',(10.,-7.47034547479885E-17,4.11));
#6714=CARTESIAN_POINT('Origin',(10.,0.,3.5));
#6715=CARTESIAN_POINT('Origin',(10.,0.,3.5));
#6716=CARTESIAN_POINT('',(10.,-2.44929359829471E-16,5.5));
#6717=CARTESIAN_POINT('',(10.,-2.44929359829471E-16,5.5));
#6718=CARTESIAN_POINT('Origin',(10.,0.,3.5));
#6719=CARTESIAN_POINT('Origin',(10.,0.,3.5));
#7312=UNCERTAINTY_MEASURE_WITH_UNIT(LENGTH_MEASURE(0.001),#7350,
'DISTANCE_ACCURACY_VALUE',
'Maximum model space distance between geometric entities at asserted c
onnectivities');
#7324=UNCERTAINTY_MEASURE_WITH_UNIT(LENGTH_MEASURE(0.001),#7350,
'DISTANCE_ACCURACY_VALUE',
'Maximum model space distance between geometric entities at asserted c
onnectivities');
#7337=(
GEOMETRIC_REPRESENTATION_CONTEXT(3)
GLOBAL_UNCERTAINTY_ASSIGNED_CONTEXT((#7312))
GLOBAL_UNIT_ASSIGNED_CONTEXT((#7350,#7352,#7353))
REPRESENTATION_CONTEXT('','3D')
);
#7349=(
GEOMETRIC_REPRESENTATION_CONTEXT(3)
GLOBAL_UNCERTAINTY_ASSIGNED_CONTEXT((#7324))
GLOBAL_UNIT_ASSIGNED_CONTEXT((#7350,#7352,#7353))
REPRESENTATION_CONTEXT('','3D')
);
#7350=(
LENGTH_UNIT()
NAMED_UNIT(*)
SI_UNIT(.CENTI.,.METRE.)
);
#7352=(
NAMED_UNIT(*)
PLANE_ANGLE_UNIT()
SI_UNIT($,.RADIAN.)
);
#7353=(
NAMED_UNIT(*)
SI_UNIT($,.STERADIAN.)
SOLID_ANGLE_UNIT()
);
#7366=SHAPE_DEFINITION_REPRESENTATION(#7390,#7453);
#7390=PRODUCT_DEFINITION_SHAPE('',$,#7478);
#7453=SHAPE_REPRESENTATION('',(#4446),#7337);
#7465=PRODUCT_DEFINITION_CONTEXT('part definition',#7539,'design');
#7478=PRODUCT_DEFINITION('Split locking cap','Split locking cap',#7502,
#7465);
#7502=PRODUCT_DEFINITION_FORMATION('',$,#7553);
#7539=APPLICATION_CONTEXT(
'Core Data for Automotive Mechanical Design Process');
#7540=PRODUCT_CONTEXT('part definition',#7539,'mechanical');
#7553=PRODUCT('Split locking cap','Split locking cap',
'Split locking cap',(#7540));
#7614=COLOUR_RGB('Sky Blue',0.24,0.69,0.87);
#7615=FILL_AREA_STYLE_COLOUR('',#7614);
#7616=FILL_AREA_STYLE('',(#7615));
#7617=SURFACE_STYLE_FILL_AREA(#7616);
#7618=SURFACE_SIDE_STYLE('',(#7617));
#7619=SURFACE_STYLE_USAGE(.BOTH.,#7618);
#7620=PRESENTATION_STYLE_ASSIGNMENT((#7619));
ENDSEC;
END-ISO-10303-21;
